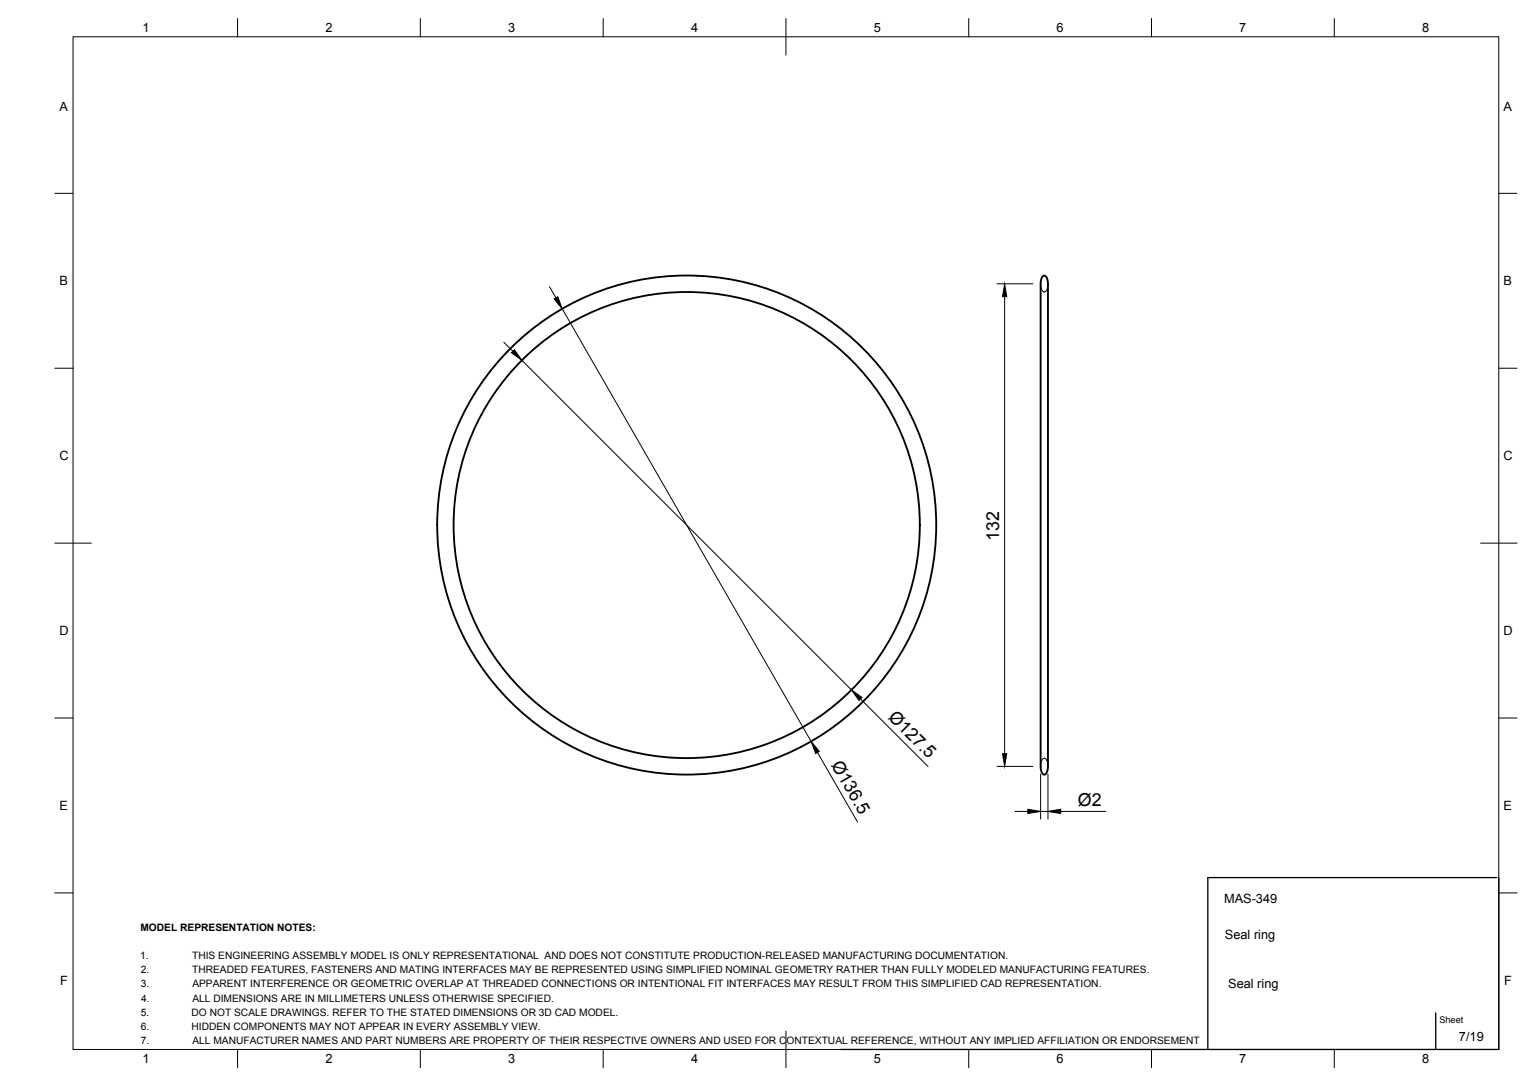
ISO-10303-21;
HEADER;
/* Generated by software containing ST-Developer
 * from STEP Tools, Inc. (www.steptools.com) 
 */

FILE_DESCRIPTION(
/* description */ ('Independent two-stage semi-open centrifugal-pump CAD. Shared impeller
s, open-machinable return casings, removable diaphragms, bronze wear/j
ournal rings, volume-preserving seal instances, retained keyed shaft, 
opposed mechanical face rings and partly threaded tie hardware. Native
 shaft rotation. Geometric topology/clearance only; flow/head/efficien
cy, pressure, cavitation, balance, preload, face loading and secondary
 seal fits/bonds, material/thermal/tolerance selection and life unassi
gned. External drive, coupling, anchors and piping bolts omitted.'),
/* implementation_level */ '2;1');

FILE_NAME(
/* name */ 'Seal ring.step',
/* time_stamp */ '2026-11-08T18:06:32-08:00',
/* author */ (''),
/* organization */ (''),
/* preprocessor_version */ 'ST-DEVELOPER v20.2',
/* originating_system */ 'Autodesk Translation Framework v15.17.0.0',
/* authorisation */ '');

FILE_SCHEMA (('AUTOMOTIVE_DESIGN { 1 0 10303 214 3 1 1 }'));
ENDSEC;

DATA;
#10=MECHANICAL_DESIGN_GEOMETRIC_PRESENTATION_REPRESENTATION('',(#398),#16687);
#136=ELLIPSE('',#6713,0.225,0.1);
#137=(
BOUNDED_SURFACE()
B_SPLINE_SURFACE(2,2,((#14548,#14549,#14550,#14551,#14552,#14553,#14554,
#14555,#14556),(#14557,#14558,#14559,#14560,#14561,#14562,#14563,#14564,
#14565),(#14566,#14567,#14568,#14569,#14570,#14571,#14572,#14573,#14574),
(#14575,#14576,#14577,#14578,#14579,#14580,#14581,#14582,#14583),(#14584,
#14585,#14586,#14587,#14588,#14589,#14590,#14591,#14592),(#14593,#14594,
#14595,#14596,#14597,#14598,#14599,#14600,#14601),(#14602,#14603,#14604,
#14605,#14606,#14607,#14608,#14609,#14610),(#14611,#14612,#14613,#14614,
#14615,#14616,#14617,#14618,#14619),(#14620,#14621,#14622,#14623,#14624,
#14625,#14626,#14627,#14628)),.UNSPECIFIED.,.T.,.T.,.F.)
B_SPLINE_SURFACE_WITH_KNOTS((3,2,2,2,3),(3,2,2,2,3),(-3.14159265358979,
-1.5707963267949,0.,1.5707963267949,3.14159265358979),(0.,1.5707963267949,
3.14159265358979,4.71238898038469,6.28318530717959),.UNSPECIFIED.)
GEOMETRIC_REPRESENTATION_ITEM()
RATIONAL_B_SPLINE_SURFACE(((1.,0.707106781186548,1.,0.707106781186548,1.,
0.707106781186548,1.,0.707106781186548,1.),(0.707106781186547,0.5,0.707106781186547,
0.5,0.707106781186547,0.5,0.707106781186547,0.5,0.707106781186547),(1.,
0.707106781186548,1.,0.707106781186548,1.,0.707106781186548,1.,0.707106781186548,
1.),(0.707106781186547,0.499999999999999,0.707106781186547,0.499999999999999,
0.707106781186547,0.499999999999999,0.707106781186547,0.499999999999999,
0.707106781186547),(1.,0.707106781186548,1.,0.707106781186548,1.,0.707106781186548,
1.,0.707106781186548,1.),(0.707106781186547,0.499999999999999,0.707106781186547,
0.499999999999999,0.707106781186547,0.499999999999999,0.707106781186547,
0.499999999999999,0.707106781186547),(1.,0.707106781186548,1.,0.707106781186548,
1.,0.707106781186548,1.,0.707106781186548,1.),(0.707106781186546,0.499999999999999,
0.707106781186546,0.499999999999999,0.707106781186546,0.499999999999999,
0.707106781186546,0.499999999999999,0.707106781186546),(1.,0.707106781186548,
1.,0.707106781186548,1.,0.707106781186548,1.,0.707106781186548,1.)))
REPRESENTATION_ITEM('')
SURFACE()
);
#360=SHAPE_REPRESENTATION_RELATIONSHIP('SRR','None',#16769,#379);
#379=ADVANCED_BREP_SHAPE_REPRESENTATION('',(#417),#16673);
#398=STYLED_ITEM('',(#16872),#417);
#417=MANIFOLD_SOLID_BREP('Body1',#6117);
#903=FACE_OUTER_BOUND('',#1322,.T.);
#1322=EDGE_LOOP('',(#5025,#5026,#5027,#5028));
#2396=CIRCLE('',#6714,6.375);
#2877=VERTEX_POINT('',#14629);
#3622=EDGE_CURVE('',#2877,#2877,#136,.T.);
#3623=EDGE_CURVE('',#2877,#2877,#2396,.T.);
#5025=ORIENTED_EDGE('',*,*,#3622,.T.);
#5026=ORIENTED_EDGE('',*,*,#3623,.T.);
#5027=ORIENTED_EDGE('',*,*,#3622,.F.);
#5028=ORIENTED_EDGE('',*,*,#3623,.F.);
#5982=ADVANCED_FACE('',(#903),#137,.T.);
#6117=CLOSED_SHELL('',(#5982));
#6712=AXIS2_PLACEMENT_3D('',#14547,#7981,#7982);
#6713=AXIS2_PLACEMENT_3D('',#14630,#7983,#7984);
#6714=AXIS2_PLACEMENT_3D('',#14631,#7985,#7986);
#7981=DIRECTION('axis',(0.,0.,1.));
#7982=DIRECTION('refdir',(1.,0.,0.));
#7983=DIRECTION('center_axis',(0.,1.,0.));
#7984=DIRECTION('ref_axis',(1.,0.,0.));
#7985=DIRECTION('center_axis',(0.,0.,1.));
#7986=DIRECTION('ref_axis',(1.,0.,0.));
#14547=CARTESIAN_POINT('',(0.,0.,0.));
#14548=CARTESIAN_POINT('Ctrl Pts',(6.375,0.,-0.1));
#14549=CARTESIAN_POINT('Ctrl Pts',(6.375,6.375,-0.1));
#14550=CARTESIAN_POINT('Ctrl Pts',(0.,6.375,-0.1));
#14551=CARTESIAN_POINT('Ctrl Pts',(-6.375,6.375,-0.1));
#14552=CARTESIAN_POINT('Ctrl Pts',(-6.375,0.,-0.1));
#14553=CARTESIAN_POINT('Ctrl Pts',(-6.375,-6.375,-0.1));
#14554=CARTESIAN_POINT('Ctrl Pts',(0.,-6.375,-0.1));
#14555=CARTESIAN_POINT('Ctrl Pts',(6.375,-6.375,-0.1));
#14556=CARTESIAN_POINT('Ctrl Pts',(6.375,0.,-0.1));
#14557=CARTESIAN_POINT('Ctrl Pts',(6.375,0.,3.06161699786838E-18));
#14558=CARTESIAN_POINT('Ctrl Pts',(6.375,6.375,3.06161699786838E-18));
#14559=CARTESIAN_POINT('Ctrl Pts',(0.,6.375,0.));
#14560=CARTESIAN_POINT('Ctrl Pts',(-6.375,6.375,-3.06161699786838E-18));
#14561=CARTESIAN_POINT('Ctrl Pts',(-6.375,0.,-3.06161699786838E-18));
#14562=CARTESIAN_POINT('Ctrl Pts',(-6.375,-6.375,-3.06161699786838E-18));
#14563=CARTESIAN_POINT('Ctrl Pts',(0.,-6.375,0.));
#14564=CARTESIAN_POINT('Ctrl Pts',(6.375,-6.375,3.06161699786838E-18));
#14565=CARTESIAN_POINT('Ctrl Pts',(6.375,0.,3.06161699786838E-18));
#14566=CARTESIAN_POINT('Ctrl Pts',(6.6,0.,0.));
#14567=CARTESIAN_POINT('Ctrl Pts',(6.6,6.6,0.));
#14568=CARTESIAN_POINT('Ctrl Pts',(0.,6.6,0.));
#14569=CARTESIAN_POINT('Ctrl Pts',(-6.6,6.6,0.));
#14570=CARTESIAN_POINT('Ctrl Pts',(-6.6,0.,0.));
#14571=CARTESIAN_POINT('Ctrl Pts',(-6.6,-6.6,0.));
#14572=CARTESIAN_POINT('Ctrl Pts',(0.,-6.6,0.));
#14573=CARTESIAN_POINT('Ctrl Pts',(6.6,-6.6,0.));
#14574=CARTESIAN_POINT('Ctrl Pts',(6.6,0.,0.));
#14575=CARTESIAN_POINT('Ctrl Pts',(6.825,0.,-3.06161699786838E-18));
#14576=CARTESIAN_POINT('Ctrl Pts',(6.825,6.825,-3.06161699786838E-18));
#14577=CARTESIAN_POINT('Ctrl Pts',(0.,6.825,0.));
#14578=CARTESIAN_POINT('Ctrl Pts',(-6.825,6.825,3.06161699786838E-18));
#14579=CARTESIAN_POINT('Ctrl Pts',(-6.825,0.,3.06161699786838E-18));
#14580=CARTESIAN_POINT('Ctrl Pts',(-6.825,-6.825,3.06161699786838E-18));
#14581=CARTESIAN_POINT('Ctrl Pts',(0.,-6.825,0.));
#14582=CARTESIAN_POINT('Ctrl Pts',(6.825,-6.825,-3.06161699786838E-18));
#14583=CARTESIAN_POINT('Ctrl Pts',(6.825,0.,-3.06161699786838E-18));
#14584=CARTESIAN_POINT('Ctrl Pts',(6.825,0.,-0.1));
#14585=CARTESIAN_POINT('Ctrl Pts',(6.825,6.825,-0.1));
#14586=CARTESIAN_POINT('Ctrl Pts',(0.,6.825,-0.1));
#14587=CARTESIAN_POINT('Ctrl Pts',(-6.825,6.825,-0.1));
#14588=CARTESIAN_POINT('Ctrl Pts',(-6.825,0.,-0.1));
#14589=CARTESIAN_POINT('Ctrl Pts',(-6.825,-6.825,-0.1));
#14590=CARTESIAN_POINT('Ctrl Pts',(0.,-6.825,-0.1));
#14591=CARTESIAN_POINT('Ctrl Pts',(6.825,-6.825,-0.1));
#14592=CARTESIAN_POINT('Ctrl Pts',(6.825,0.,-0.1));
#14593=CARTESIAN_POINT('Ctrl Pts',(6.825,0.,-0.2));
#14594=CARTESIAN_POINT('Ctrl Pts',(6.825,6.825,-0.2));
#14595=CARTESIAN_POINT('Ctrl Pts',(0.,6.825,-0.2));
#14596=CARTESIAN_POINT('Ctrl Pts',(-6.825,6.825,-0.2));
#14597=CARTESIAN_POINT('Ctrl Pts',(-6.825,0.,-0.2));
#14598=CARTESIAN_POINT('Ctrl Pts',(-6.825,-6.825,-0.2));
#14599=CARTESIAN_POINT('Ctrl Pts',(0.,-6.825,-0.2));
#14600=CARTESIAN_POINT('Ctrl Pts',(6.825,-6.825,-0.2));
#14601=CARTESIAN_POINT('Ctrl Pts',(6.825,0.,-0.2));
#14602=CARTESIAN_POINT('Ctrl Pts',(6.6,0.,-0.2));
#14603=CARTESIAN_POINT('Ctrl Pts',(6.6,6.6,-0.2));
#14604=CARTESIAN_POINT('Ctrl Pts',(0.,6.6,-0.2));
#14605=CARTESIAN_POINT('Ctrl Pts',(-6.6,6.6,-0.2));
#14606=CARTESIAN_POINT('Ctrl Pts',(-6.6,0.,-0.2));
#14607=CARTESIAN_POINT('Ctrl Pts',(-6.6,-6.6,-0.2));
#14608=CARTESIAN_POINT('Ctrl Pts',(0.,-6.6,-0.2));
#14609=CARTESIAN_POINT('Ctrl Pts',(6.6,-6.6,-0.2));
#14610=CARTESIAN_POINT('Ctrl Pts',(6.6,0.,-0.2));
#14611=CARTESIAN_POINT('Ctrl Pts',(6.375,0.,-0.2));
#14612=CARTESIAN_POINT('Ctrl Pts',(6.375,6.375,-0.2));
#14613=CARTESIAN_POINT('Ctrl Pts',(0.,6.375,-0.2));
#14614=CARTESIAN_POINT('Ctrl Pts',(-6.375,6.375,-0.2));
#14615=CARTESIAN_POINT('Ctrl Pts',(-6.375,0.,-0.2));
#14616=CARTESIAN_POINT('Ctrl Pts',(-6.375,-6.375,-0.2));
#14617=CARTESIAN_POINT('Ctrl Pts',(0.,-6.375,-0.2));
#14618=CARTESIAN_POINT('Ctrl Pts',(6.375,-6.375,-0.2));
#14619=CARTESIAN_POINT('Ctrl Pts',(6.375,0.,-0.2));
#14620=CARTESIAN_POINT('Ctrl Pts',(6.375,0.,-0.1));
#14621=CARTESIAN_POINT('Ctrl Pts',(6.375,6.375,-0.1));
#14622=CARTESIAN_POINT('Ctrl Pts',(0.,6.375,-0.1));
#14623=CARTESIAN_POINT('Ctrl Pts',(-6.375,6.375,-0.1));
#14624=CARTESIAN_POINT('Ctrl Pts',(-6.375,0.,-0.1));
#14625=CARTESIAN_POINT('Ctrl Pts',(-6.375,-6.375,-0.1));
#14626=CARTESIAN_POINT('Ctrl Pts',(0.,-6.375,-0.1));
#14627=CARTESIAN_POINT('Ctrl Pts',(6.375,-6.375,-0.1));
#14628=CARTESIAN_POINT('Ctrl Pts',(6.375,0.,-0.1));
#14629=CARTESIAN_POINT('',(6.375,0.,-0.1));
#14630=CARTESIAN_POINT('Origin',(6.6,0.,-0.1));
#14631=CARTESIAN_POINT('Origin',(0.,0.,-0.1));
#16652=UNCERTAINTY_MEASURE_WITH_UNIT(LENGTH_MEASURE(0.001),#16688,
'DISTANCE_ACCURACY_VALUE',
'Maximum model space distance between geometric entities at asserted c
onnectivities');
#16666=UNCERTAINTY_MEASURE_WITH_UNIT(LENGTH_MEASURE(0.001),#16688,
'DISTANCE_ACCURACY_VALUE',
'Maximum model space distance between geometric entities at asserted c
onnectivities');
#16673=(
GEOMETRIC_REPRESENTATION_CONTEXT(3)
GLOBAL_UNCERTAINTY_ASSIGNED_CONTEXT((#16652))
GLOBAL_UNIT_ASSIGNED_CONTEXT((#16688,#16690,#16691))
REPRESENTATION_CONTEXT('','3D')
);
#16687=(
GEOMETRIC_REPRESENTATION_CONTEXT(3)
GLOBAL_UNCERTAINTY_ASSIGNED_CONTEXT((#16666))
GLOBAL_UNIT_ASSIGNED_CONTEXT((#16688,#16690,#16691))
REPRESENTATION_CONTEXT('','3D')
);
#16688=(
LENGTH_UNIT()
NAMED_UNIT(*)
SI_UNIT(.CENTI.,.METRE.)
);
#16690=(
NAMED_UNIT(*)
PLANE_ANGLE_UNIT()
SI_UNIT($,.RADIAN.)
);
#16691=(
NAMED_UNIT(*)
SI_UNIT($,.STERADIAN.)
SOLID_ANGLE_UNIT()
);
#16698=SHAPE_DEFINITION_REPRESENTATION(#16718,#16769);
#16718=PRODUCT_DEFINITION_SHAPE('',$,#16790);
#16769=SHAPE_REPRESENTATION('',(#6712),#16673);
#16783=PRODUCT_DEFINITION_CONTEXT('part definition',#16845,'design');
#16790=PRODUCT_DEFINITION('Seal ring','Seal ring',#16810,#16783);
#16810=PRODUCT_DEFINITION_FORMATION('',$,#16853);
#16845=APPLICATION_CONTEXT(
'Core Data for Automotive Mechanical Design Process');
#16846=PRODUCT_CONTEXT('part definition',#16845,'mechanical');
#16853=PRODUCT('Seal ring','Seal ring',
'Reusable132mm mean-diameter ring,3mm circular free wire,2mm installed
 axial height and derived4.5mm radial width preserving cross-section a
rea. Native constrained ellipse and revolve; gland/material/pressure s
election unassigned.',(#16846));
#16872=PRESENTATION_STYLE_ASSIGNMENT((#16887));
#16887=SURFACE_STYLE_USAGE(.BOTH.,#16902);
#16902=SURFACE_SIDE_STYLE('',(#16917));
#16917=SURFACE_STYLE_FILL_AREA(#16932);
#16932=FILL_AREA_STYLE('Seal charcoal',(#16947));
#16947=FILL_AREA_STYLE_COLOUR('Seal charcoal',#16962);
#16962=COLOUR_RGB('Seal charcoal',0.164705882352941,0.184313725490196,0.211764705882353);
ENDSEC;
END-ISO-10303-21;
